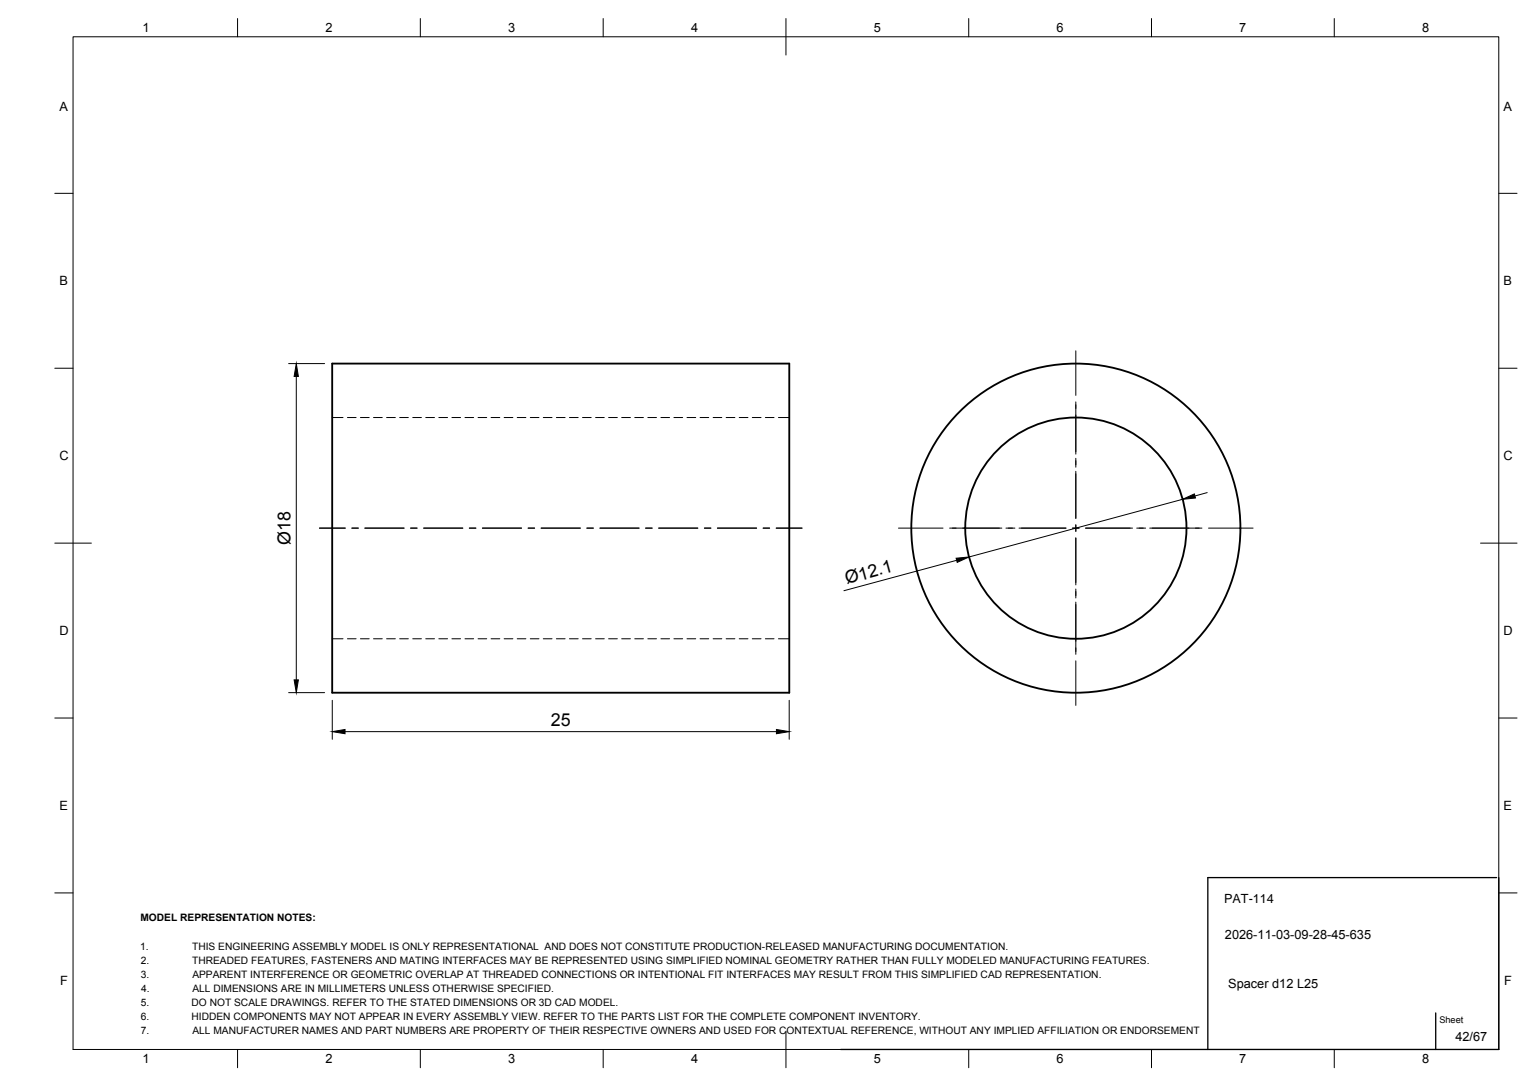
ISO-10303-21;
HEADER;
/* Generated by software containing ST-Developer
 * from STEP Tools, Inc. (www.steptools.com) 
 */

FILE_DESCRIPTION(
/* description */ ('Two-stage gear reducer in split housing'),
/* implementation_level */ '2;1');

FILE_NAME(
/* name */ 'Spacer d12 L25.step',
/* time_stamp */ '2026-10-28T03:22:31-07:00',
/* author */ (''),
/* organization */ (''),
/* preprocessor_version */ 'ST-DEVELOPER v20.2',
/* originating_system */ 'Autodesk Translation Framework v15.17.0.0',
/* authorisation */ '');

FILE_SCHEMA (('AUTOMOTIVE_DESIGN { 1 0 10303 214 3 1 1 }'));
ENDSEC;

DATA;
#10=MECHANICAL_DESIGN_GEOMETRIC_PRESENTATION_REPRESENTATION('',(#1282),#73366);
#1155=SHAPE_REPRESENTATION_RELATIONSHIP('SRR','None',#73645,#1211);
#1211=ADVANCED_BREP_SHAPE_REPRESENTATION('',(#1351),#73341);
#1282=STYLED_ITEM('',(#74002),#1351);
#1351=MANIFOLD_SOLID_BREP('Body1',#16172);
#1551=FACE_BOUND('',#3539,.T.);
#1552=FACE_BOUND('',#3541,.T.);
#1818=PLANE('',#17833);
#1819=PLANE('',#17834);
#2446=FACE_OUTER_BOUND('',#3536,.T.);
#2447=FACE_OUTER_BOUND('',#3537,.T.);
#2448=FACE_OUTER_BOUND('',#3538,.T.);
#2449=FACE_OUTER_BOUND('',#3540,.T.);
#3536=EDGE_LOOP('',(#12407,#12408,#12409,#12410));
#3537=EDGE_LOOP('',(#12411,#12412,#12413,#12414));
#3538=EDGE_LOOP('',(#12415));
#3539=EDGE_LOOP('',(#12416));
#3540=EDGE_LOOP('',(#12417));
#3541=EDGE_LOOP('',(#12418));
#4504=LINE('',#25666,#5528);
#4505=LINE('',#25672,#5529);
#5528=VECTOR('',#20940,0.605);
#5529=VECTOR('',#20947,0.9);
#6566=CIRCLE('',#17828,0.605);
#6567=CIRCLE('',#17829,0.605);
#6568=CIRCLE('',#17831,0.9);
#6569=CIRCLE('',#17832,0.9);
#7473=VERTEX_POINT('',#25663);
#7474=VERTEX_POINT('',#25665);
#7475=VERTEX_POINT('',#25669);
#7476=VERTEX_POINT('',#25671);
#9257=EDGE_CURVE('',#7473,#7473,#6566,.T.);
#9258=EDGE_CURVE('',#7473,#7474,#4504,.T.);
#9259=EDGE_CURVE('',#7474,#7474,#6567,.T.);
#9260=EDGE_CURVE('',#7475,#7475,#6568,.T.);
#9261=EDGE_CURVE('',#7475,#7476,#4505,.T.);
#9262=EDGE_CURVE('',#7476,#7476,#6569,.T.);
#12407=ORIENTED_EDGE('',*,*,#9257,.F.);
#12408=ORIENTED_EDGE('',*,*,#9258,.T.);
#12409=ORIENTED_EDGE('',*,*,#9259,.T.);
#12410=ORIENTED_EDGE('',*,*,#9258,.F.);
#12411=ORIENTED_EDGE('',*,*,#9260,.F.);
#12412=ORIENTED_EDGE('',*,*,#9261,.T.);
#12413=ORIENTED_EDGE('',*,*,#9262,.T.);
#12414=ORIENTED_EDGE('',*,*,#9261,.F.);
#12415=ORIENTED_EDGE('',*,*,#9260,.T.);
#12416=ORIENTED_EDGE('',*,*,#9257,.T.);
#12417=ORIENTED_EDGE('',*,*,#9262,.F.);
#12418=ORIENTED_EDGE('',*,*,#9259,.F.);
#15086=CYLINDRICAL_SURFACE('',#17827,0.605);
#15087=CYLINDRICAL_SURFACE('',#17830,0.9);
#15653=ADVANCED_FACE('',(#2446),#15086,.F.);
#15654=ADVANCED_FACE('',(#2447),#15087,.T.);
#15655=ADVANCED_FACE('',(#2448,#1551),#1818,.T.);
#15656=ADVANCED_FACE('',(#2449,#1552),#1819,.F.);
#16172=CLOSED_SHELL('',(#15653,#15654,#15655,#15656));
#17826=AXIS2_PLACEMENT_3D('',#25661,#20934,#20935);
#17827=AXIS2_PLACEMENT_3D('',#25662,#20936,#20937);
#17828=AXIS2_PLACEMENT_3D('',#25664,#20938,#20939);
#17829=AXIS2_PLACEMENT_3D('',#25667,#20941,#20942);
#17830=AXIS2_PLACEMENT_3D('',#25668,#20943,#20944);
#17831=AXIS2_PLACEMENT_3D('',#25670,#20945,#20946);
#17832=AXIS2_PLACEMENT_3D('',#25673,#20948,#20949);
#17833=AXIS2_PLACEMENT_3D('',#25674,#20950,#20951);
#17834=AXIS2_PLACEMENT_3D('',#25675,#20952,#20953);
#20934=DIRECTION('axis',(0.,0.,1.));
#20935=DIRECTION('refdir',(1.,0.,0.));
#20936=DIRECTION('center_axis',(0.,1.,0.));
#20937=DIRECTION('ref_axis',(1.,0.,0.));
#20938=DIRECTION('center_axis',(0.,-1.,0.));
#20939=DIRECTION('ref_axis',(1.,0.,0.));
#20940=DIRECTION('',(0.,-1.,0.));
#20941=DIRECTION('center_axis',(0.,-1.,0.));
#20942=DIRECTION('ref_axis',(1.,0.,0.));
#20943=DIRECTION('center_axis',(0.,1.,0.));
#20944=DIRECTION('ref_axis',(1.,0.,0.));
#20945=DIRECTION('center_axis',(0.,1.,0.));
#20946=DIRECTION('ref_axis',(1.,0.,0.));
#20947=DIRECTION('',(0.,-1.,0.));
#20948=DIRECTION('center_axis',(0.,1.,0.));
#20949=DIRECTION('ref_axis',(1.,0.,0.));
#20950=DIRECTION('center_axis',(0.,1.,0.));
#20951=DIRECTION('ref_axis',(1.,0.,0.));
#20952=DIRECTION('center_axis',(0.,1.,0.));
#20953=DIRECTION('ref_axis',(1.,0.,0.));
#25661=CARTESIAN_POINT('',(0.,0.,0.));
#25662=CARTESIAN_POINT('Origin',(0.,-5.5,10.));
#25663=CARTESIAN_POINT('',(-0.605,-3.,10.));
#25664=CARTESIAN_POINT('Origin',(0.,-3.,10.));
#25665=CARTESIAN_POINT('',(-0.605,-5.5,10.));
#25666=CARTESIAN_POINT('',(-0.605,-5.5,10.));
#25667=CARTESIAN_POINT('Origin',(0.,-5.5,10.));
#25668=CARTESIAN_POINT('Origin',(0.,-5.5,10.));
#25669=CARTESIAN_POINT('',(-0.9,-3.,10.));
#25670=CARTESIAN_POINT('Origin',(0.,-3.,10.));
#25671=CARTESIAN_POINT('',(-0.9,-5.5,10.));
#25672=CARTESIAN_POINT('',(-0.9,-5.5,10.));
#25673=CARTESIAN_POINT('Origin',(0.,-5.5,10.));
#25674=CARTESIAN_POINT('Origin',(0.,-3.,10.));
#25675=CARTESIAN_POINT('Origin',(0.,-5.5,10.));
#73277=UNCERTAINTY_MEASURE_WITH_UNIT(LENGTH_MEASURE(0.001),#73367,
'DISTANCE_ACCURACY_VALUE',
'Maximum model space distance between geometric entities at asserted c
onnectivities');
#73302=UNCERTAINTY_MEASURE_WITH_UNIT(LENGTH_MEASURE(0.001),#73367,
'DISTANCE_ACCURACY_VALUE',
'Maximum model space distance between geometric entities at asserted c
onnectivities');
#73341=(
GEOMETRIC_REPRESENTATION_CONTEXT(3)
GLOBAL_UNCERTAINTY_ASSIGNED_CONTEXT((#73277))
GLOBAL_UNIT_ASSIGNED_CONTEXT((#73367,#73369,#73370))
REPRESENTATION_CONTEXT('','3D')
);
#73366=(
GEOMETRIC_REPRESENTATION_CONTEXT(3)
GLOBAL_UNCERTAINTY_ASSIGNED_CONTEXT((#73302))
GLOBAL_UNIT_ASSIGNED_CONTEXT((#73367,#73369,#73370))
REPRESENTATION_CONTEXT('','3D')
);
#73367=(
LENGTH_UNIT()
NAMED_UNIT(*)
SI_UNIT(.CENTI.,.METRE.)
);
#73369=(
NAMED_UNIT(*)
PLANE_ANGLE_UNIT()
SI_UNIT($,.RADIAN.)
);
#73370=(
NAMED_UNIT(*)
SI_UNIT($,.STERADIAN.)
SOLID_ANGLE_UNIT()
);
#73409=SHAPE_DEFINITION_REPRESENTATION(#73542,#73645);
#73542=PRODUCT_DEFINITION_SHAPE('',$,#73709);
#73645=SHAPE_REPRESENTATION('',(#17826),#73341);
#73670=PRODUCT_DEFINITION_CONTEXT('part definition',#73861,'design');
#73709=PRODUCT_DEFINITION('Spacer d12 L25','Spacer d12 L25',#73772,#73670);
#73772=PRODUCT_DEFINITION_FORMATION('',$,#73901);
#73861=APPLICATION_CONTEXT(
'Core Data for Automotive Mechanical Design Process');
#73862=PRODUCT_CONTEXT('part definition',#73861,'mechanical');
#73901=PRODUCT('Spacer d12 L25','Spacer d12 L25','Spacer d12 L25',(#73862));
#73996=COLOUR_RGB('Off White',0.89,0.88,0.83);
#73997=FILL_AREA_STYLE_COLOUR('',#73996);
#73998=FILL_AREA_STYLE('',(#73997));
#73999=SURFACE_STYLE_FILL_AREA(#73998);
#74000=SURFACE_SIDE_STYLE('',(#73999));
#74001=SURFACE_STYLE_USAGE(.BOTH.,#74000);
#74002=PRESENTATION_STYLE_ASSIGNMENT((#74001));
ENDSEC;
END-ISO-10303-21;
